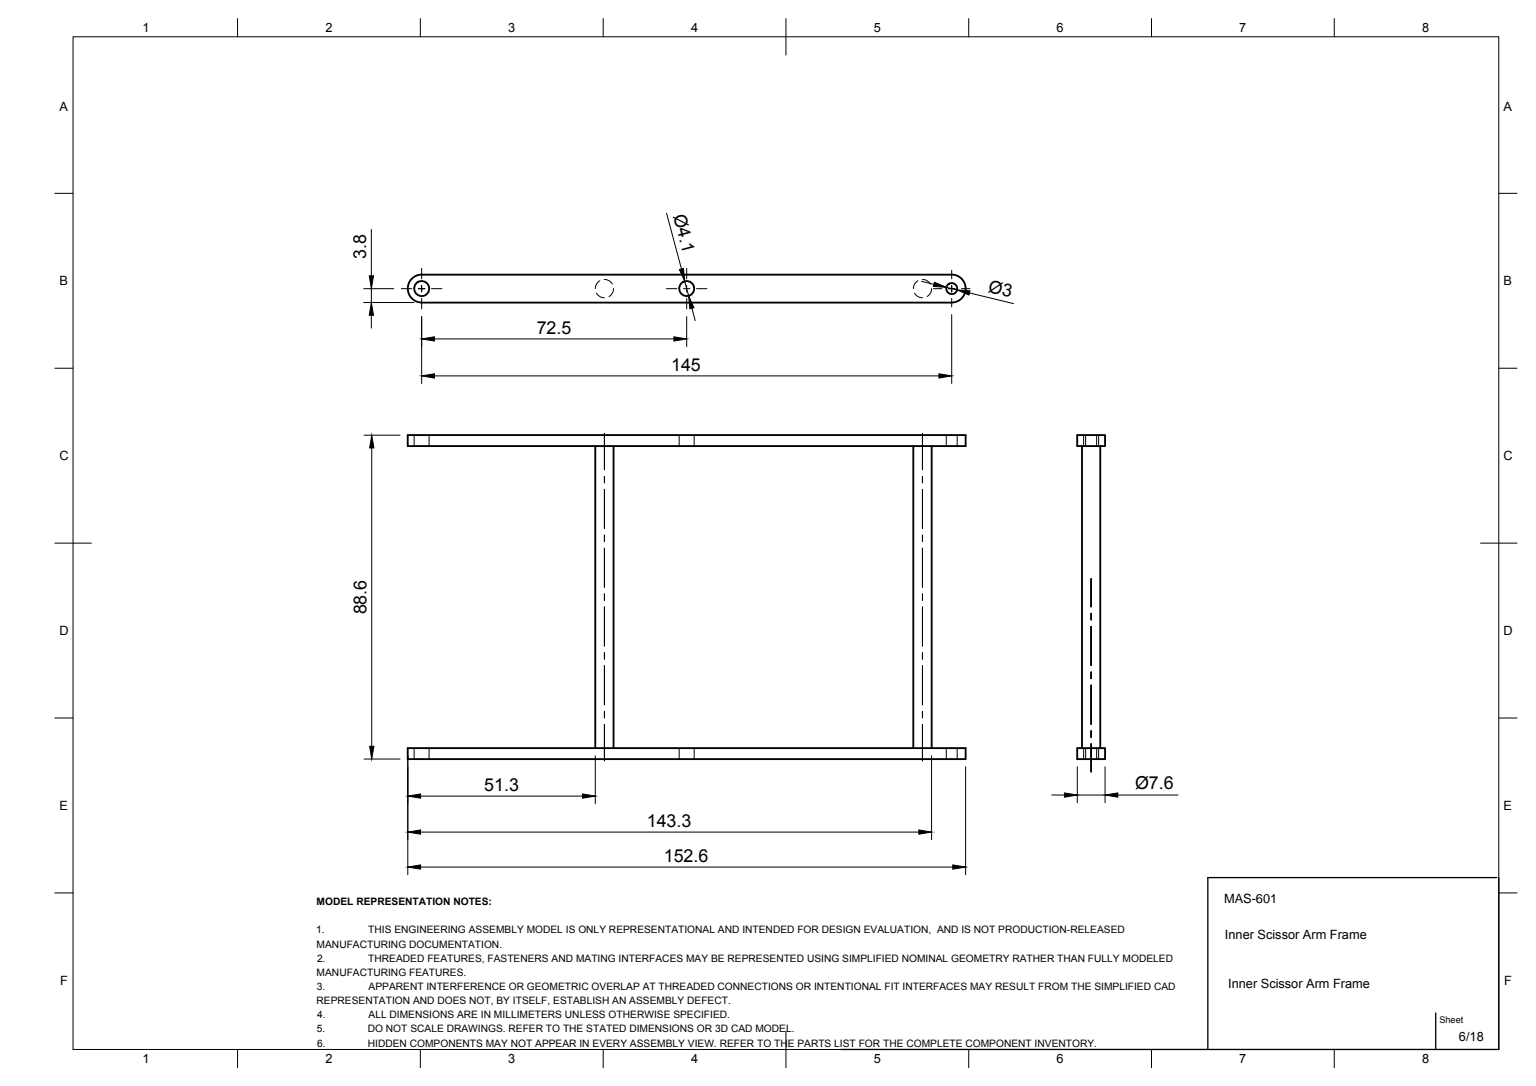
ISO-10303-21;
HEADER;
FILE_DESCRIPTION((''),'2;1');
FILE_NAME('Inner Scissor Arm Frame.step','2026-10-06T07:37:42+05:00',(''),(''),'','','');
FILE_SCHEMA (('AUTOMOTIVE_DESIGN { 1 0 10303 214 3 1 1 }'));
ENDSEC;
DATA;
#10=MECHANICAL_DESIGN_GEOMETRIC_PRESENTATION_REPRESENTATION('',(#376),#18757);
#342=SHAPE_REPRESENTATION_RELATIONSHIP('SRR','None',#18860,#359) ;
#359=ADVANCED_BREP_SHAPE_REPRESENTATION('',(#393),#18743) ;
#376=STYLED_ITEM('',(#18954),#393) ;
#393=MANIFOLD_SOLID_BREP('Inner Scissor Arm Frame',#9545) ;
#549=CYLINDRICAL_SURFACE('',#10026,2.5) ;
#550=CYLINDRICAL_SURFACE('',#10029,2.5) ;
#551=CYLINDRICAL_SURFACE('',#10032,2.05) ;
#552=CYLINDRICAL_SURFACE('',#10035,1.5) ;
#553=CYLINDRICAL_SURFACE('',#10038,2.05) ;
#554=CYLINDRICAL_SURFACE('',#10042,3.8) ;
#555=CYLINDRICAL_SURFACE('',#10046,3.8) ;
#556=CYLINDRICAL_SURFACE('',#10051,1.5) ;
#557=CYLINDRICAL_SURFACE('',#10054,2.05) ;
#558=CYLINDRICAL_SURFACE('',#10057,2.05) ;
#559=CYLINDRICAL_SURFACE('',#10061,3.8) ;
#560=CYLINDRICAL_SURFACE('',#10065,3.8) ;
#696=FACE_BOUND('',#1819,.T.) ;
#697=FACE_BOUND('',#1820,.T.) ;
#698=FACE_BOUND('',#1821,.T.) ;
#699=FACE_BOUND('',#1822,.T.) ;
#700=FACE_BOUND('',#1823,.T.) ;
#701=FACE_BOUND('',#1825,.T.) ;
#702=FACE_BOUND('',#1826,.T.) ;
#703=FACE_BOUND('',#1827,.T.) ;
#704=FACE_BOUND('',#1836,.T.) ;
#705=FACE_BOUND('',#1837,.T.) ;
#706=FACE_BOUND('',#1838,.T.) ;
#707=FACE_BOUND('',#1840,.T.) ;
#708=FACE_BOUND('',#1841,.T.) ;
#709=FACE_BOUND('',#1842,.T.) ;
#710=FACE_BOUND('',#1843,.T.) ;
#711=FACE_BOUND('',#1844,.T.) ;
#848=PLANE('',#10041) ;
#849=PLANE('',#10045) ;
#850=PLANE('',#10049) ;
#851=PLANE('',#10050) ;
#852=PLANE('',#10060) ;
#853=PLANE('',#10064) ;
#854=PLANE('',#10068) ;
#855=PLANE('',#10069) ;
#1245=FACE_OUTER_BOUND('',#1809,.T.) ;
#1246=FACE_OUTER_BOUND('',#1810,.T.) ;
#1247=FACE_OUTER_BOUND('',#1811,.T.) ;
#1248=FACE_OUTER_BOUND('',#1812,.T.) ;
#1249=FACE_OUTER_BOUND('',#1813,.T.) ;
#1250=FACE_OUTER_BOUND('',#1814,.T.) ;
#1251=FACE_OUTER_BOUND('',#1815,.T.) ;
#1252=FACE_OUTER_BOUND('',#1816,.T.) ;
#1253=FACE_OUTER_BOUND('',#1817,.T.) ;
#1254=FACE_OUTER_BOUND('',#1818,.T.) ;
#1255=FACE_OUTER_BOUND('',#1824,.T.) ;
#1256=FACE_OUTER_BOUND('',#1828,.T.) ;
#1257=FACE_OUTER_BOUND('',#1829,.T.) ;
#1258=FACE_OUTER_BOUND('',#1830,.T.) ;
#1259=FACE_OUTER_BOUND('',#1831,.T.) ;
#1260=FACE_OUTER_BOUND('',#1832,.T.) ;
#1261=FACE_OUTER_BOUND('',#1833,.T.) ;
#1262=FACE_OUTER_BOUND('',#1834,.T.) ;
#1263=FACE_OUTER_BOUND('',#1835,.T.) ;
#1264=FACE_OUTER_BOUND('',#1839,.T.) ;
#1809=EDGE_LOOP('',(#7161,#7162,#7163,#7164)) ;
#1810=EDGE_LOOP('',(#7165,#7166,#7167,#7168)) ;
#1811=EDGE_LOOP('',(#7169,#7170,#7171,#7172)) ;
#1812=EDGE_LOOP('',(#7173,#7174,#7175,#7176)) ;
#1813=EDGE_LOOP('',(#7177,#7178,#7179,#7180)) ;
#1814=EDGE_LOOP('',(#7181,#7182,#7183,#7184)) ;
#1815=EDGE_LOOP('',(#7185,#7186,#7187,#7188)) ;
#1816=EDGE_LOOP('',(#7189,#7190,#7191,#7192)) ;
#1817=EDGE_LOOP('',(#7193,#7194,#7195,#7196)) ;
#1818=EDGE_LOOP('',(#7197,#7198,#7199,#7200)) ;
#1819=EDGE_LOOP('',(#7201)) ;
#1820=EDGE_LOOP('',(#7202)) ;
#1821=EDGE_LOOP('',(#7203)) ;
#1822=EDGE_LOOP('',(#7204)) ;
#1823=EDGE_LOOP('',(#7205)) ;
#1824=EDGE_LOOP('',(#7206,#7207,#7208,#7209)) ;
#1825=EDGE_LOOP('',(#7210)) ;
#1826=EDGE_LOOP('',(#7211)) ;
#1827=EDGE_LOOP('',(#7212)) ;
#1828=EDGE_LOOP('',(#7213,#7214,#7215,#7216)) ;
#1829=EDGE_LOOP('',(#7217,#7218,#7219,#7220)) ;
#1830=EDGE_LOOP('',(#7221,#7222,#7223,#7224)) ;
#1831=EDGE_LOOP('',(#7225,#7226,#7227,#7228)) ;
#1832=EDGE_LOOP('',(#7229,#7230,#7231,#7232)) ;
#1833=EDGE_LOOP('',(#7233,#7234,#7235,#7236)) ;
#1834=EDGE_LOOP('',(#7237,#7238,#7239,#7240)) ;
#1835=EDGE_LOOP('',(#7241,#7242,#7243,#7244)) ;
#1836=EDGE_LOOP('',(#7245)) ;
#1837=EDGE_LOOP('',(#7246)) ;
#1838=EDGE_LOOP('',(#7247)) ;
#1839=EDGE_LOOP('',(#7248,#7249,#7250,#7251)) ;
#1840=EDGE_LOOP('',(#7252)) ;
#1841=EDGE_LOOP('',(#7253)) ;
#1842=EDGE_LOOP('',(#7254)) ;
#1843=EDGE_LOOP('',(#7255)) ;
#1844=EDGE_LOOP('',(#7256)) ;
#2514=LINE('',#14482,#3285) ;
#2515=LINE('',#14488,#3286) ;
#2516=LINE('',#14494,#3287) ;
#2517=LINE('',#14500,#3288) ;
#2518=LINE('',#14506,#3289) ;
#2519=LINE('',#14511,#3290) ;
#2520=LINE('',#14513,#3291) ;
#2521=LINE('',#14515,#3292) ;
#2522=LINE('',#14516,#3293) ;
#2523=LINE('',#14522,#3294) ;
#2524=LINE('',#14525,#3295) ;
#2525=LINE('',#14527,#3296) ;
#2526=LINE('',#14528,#3297) ;
#2527=LINE('',#14538,#3298) ;
#2528=LINE('',#14544,#3299) ;
#2529=LINE('',#14550,#3300) ;
#2530=LINE('',#14555,#3301) ;
#2531=LINE('',#14557,#3302) ;
#2532=LINE('',#14559,#3303) ;
#2533=LINE('',#14560,#3304) ;
#2534=LINE('',#14566,#3305) ;
#2535=LINE('',#14569,#3306) ;
#2536=LINE('',#14571,#3307) ;
#2537=LINE('',#14572,#3308) ;
#3285=VECTOR('',#11558,2.5) ;
#3286=VECTOR('',#11565,2.5) ;
#3287=VECTOR('',#11572,2.05) ;
#3288=VECTOR('',#11579,1.5) ;
#3289=VECTOR('',#11586,2.05) ;
#3290=VECTOR('',#11591,10.) ;
#3291=VECTOR('',#11592,10.) ;
#3292=VECTOR('',#11593,10.) ;
#3293=VECTOR('',#11594,10.) ;
#3294=VECTOR('',#11601,10.) ;
#3295=VECTOR('',#11604,10.) ;
#3296=VECTOR('',#11605,10.) ;
#3297=VECTOR('',#11606,10.) ;
#3298=VECTOR('',#11621,1.5) ;
#3299=VECTOR('',#11628,2.05) ;
#3300=VECTOR('',#11635,2.05) ;
#3301=VECTOR('',#11640,10.) ;
#3302=VECTOR('',#11641,10.) ;
#3303=VECTOR('',#11642,10.) ;
#3304=VECTOR('',#11643,10.) ;
#3305=VECTOR('',#11650,10.) ;
#3306=VECTOR('',#11653,10.) ;
#3307=VECTOR('',#11654,10.) ;
#3308=VECTOR('',#11655,10.) ;
#3891=CIRCLE('',#10027,2.5) ;
#3892=CIRCLE('',#10028,2.5) ;
#3893=CIRCLE('',#10030,2.5) ;
#3894=CIRCLE('',#10031,2.5) ;
#3895=CIRCLE('',#10033,2.05) ;
#3896=CIRCLE('',#10034,2.05) ;
#3897=CIRCLE('',#10036,1.5) ;
#3898=CIRCLE('',#10037,1.5) ;
#3899=CIRCLE('',#10039,2.05) ;
#3900=CIRCLE('',#10040,2.05) ;
#3901=CIRCLE('',#10043,3.8) ;
#3902=CIRCLE('',#10044,3.8) ;
#3903=CIRCLE('',#10047,3.8) ;
#3904=CIRCLE('',#10048,3.8) ;
#3905=CIRCLE('',#10052,1.5) ;
#3906=CIRCLE('',#10053,1.5) ;
#3907=CIRCLE('',#10055,2.05) ;
#3908=CIRCLE('',#10056,2.05) ;
#3909=CIRCLE('',#10058,2.05) ;
#3910=CIRCLE('',#10059,2.05) ;
#3911=CIRCLE('',#10062,3.8) ;
#3912=CIRCLE('',#10063,3.8) ;
#3913=CIRCLE('',#10066,3.8) ;
#3914=CIRCLE('',#10067,3.8) ;
#4418=VERTEX_POINT('',#14479) ;
#4419=VERTEX_POINT('',#14481) ;
#4420=VERTEX_POINT('',#14485) ;
#4421=VERTEX_POINT('',#14487) ;
#4422=VERTEX_POINT('',#14491) ;
#4423=VERTEX_POINT('',#14493) ;
#4424=VERTEX_POINT('',#14497) ;
#4425=VERTEX_POINT('',#14499) ;
#4426=VERTEX_POINT('',#14503) ;
#4427=VERTEX_POINT('',#14505) ;
#4428=VERTEX_POINT('',#14509) ;
#4429=VERTEX_POINT('',#14510) ;
#4430=VERTEX_POINT('',#14512) ;
#4431=VERTEX_POINT('',#14514) ;
#4432=VERTEX_POINT('',#14518) ;
#4433=VERTEX_POINT('',#14520) ;
#4434=VERTEX_POINT('',#14524) ;
#4435=VERTEX_POINT('',#14526) ;
#4436=VERTEX_POINT('',#14535) ;
#4437=VERTEX_POINT('',#14537) ;
#4438=VERTEX_POINT('',#14541) ;
#4439=VERTEX_POINT('',#14543) ;
#4440=VERTEX_POINT('',#14547) ;
#4441=VERTEX_POINT('',#14549) ;
#4442=VERTEX_POINT('',#14553) ;
#4443=VERTEX_POINT('',#14554) ;
#4444=VERTEX_POINT('',#14556) ;
#4445=VERTEX_POINT('',#14558) ;
#4446=VERTEX_POINT('',#14562) ;
#4447=VERTEX_POINT('',#14564) ;
#4448=VERTEX_POINT('',#14568) ;
#4449=VERTEX_POINT('',#14570) ;
#5427=EDGE_CURVE('',#4418,#4418,#3891,.T.) ;
#5428=EDGE_CURVE('',#4418,#4419,#2514,.T.) ;
#5429=EDGE_CURVE('',#4419,#4419,#3892,.T.) ;
#5430=EDGE_CURVE('',#4420,#4420,#3893,.T.) ;
#5431=EDGE_CURVE('',#4420,#4421,#2515,.T.) ;
#5432=EDGE_CURVE('',#4421,#4421,#3894,.T.) ;
#5433=EDGE_CURVE('',#4422,#4422,#3895,.T.) ;
#5434=EDGE_CURVE('',#4422,#4423,#2516,.T.) ;
#5435=EDGE_CURVE('',#4423,#4423,#3896,.T.) ;
#5436=EDGE_CURVE('',#4424,#4424,#3897,.T.) ;
#5437=EDGE_CURVE('',#4424,#4425,#2517,.T.) ;
#5438=EDGE_CURVE('',#4425,#4425,#3898,.T.) ;
#5439=EDGE_CURVE('',#4426,#4426,#3899,.T.) ;
#5440=EDGE_CURVE('',#4426,#4427,#2518,.T.) ;
#5441=EDGE_CURVE('',#4427,#4427,#3900,.T.) ;
#5442=EDGE_CURVE('',#4428,#4429,#2519,.T.) ;
#5443=EDGE_CURVE('',#4429,#4430,#2520,.T.) ;
#5444=EDGE_CURVE('',#4431,#4430,#2521,.T.) ;
#5445=EDGE_CURVE('',#4428,#4431,#2522,.T.) ;
#5446=EDGE_CURVE('',#4432,#4428,#3901,.T.) ;
#5447=EDGE_CURVE('',#4433,#4431,#3902,.T.) ;
#5448=EDGE_CURVE('',#4432,#4433,#2523,.T.) ;
#5449=EDGE_CURVE('',#4434,#4432,#2524,.T.) ;
#5450=EDGE_CURVE('',#4435,#4433,#2525,.T.) ;
#5451=EDGE_CURVE('',#4434,#4435,#2526,.T.) ;
#5452=EDGE_CURVE('',#4429,#4434,#3903,.T.) ;
#5453=EDGE_CURVE('',#4430,#4435,#3904,.T.) ;
#5454=EDGE_CURVE('',#4436,#4436,#3905,.T.) ;
#5455=EDGE_CURVE('',#4436,#4437,#2527,.T.) ;
#5456=EDGE_CURVE('',#4437,#4437,#3906,.T.) ;
#5457=EDGE_CURVE('',#4438,#4438,#3907,.T.) ;
#5458=EDGE_CURVE('',#4438,#4439,#2528,.T.) ;
#5459=EDGE_CURVE('',#4439,#4439,#3908,.T.) ;
#5460=EDGE_CURVE('',#4440,#4440,#3909,.T.) ;
#5461=EDGE_CURVE('',#4440,#4441,#2529,.T.) ;
#5462=EDGE_CURVE('',#4441,#4441,#3910,.T.) ;
#5463=EDGE_CURVE('',#4442,#4443,#2530,.T.) ;
#5464=EDGE_CURVE('',#4443,#4444,#2531,.T.) ;
#5465=EDGE_CURVE('',#4445,#4444,#2532,.T.) ;
#5466=EDGE_CURVE('',#4442,#4445,#2533,.T.) ;
#5467=EDGE_CURVE('',#4446,#4442,#3911,.T.) ;
#5468=EDGE_CURVE('',#4447,#4445,#3912,.T.) ;
#5469=EDGE_CURVE('',#4446,#4447,#2534,.T.) ;
#5470=EDGE_CURVE('',#4448,#4446,#2535,.T.) ;
#5471=EDGE_CURVE('',#4449,#4447,#2536,.T.) ;
#5472=EDGE_CURVE('',#4448,#4449,#2537,.T.) ;
#5473=EDGE_CURVE('',#4443,#4448,#3913,.T.) ;
#5474=EDGE_CURVE('',#4444,#4449,#3914,.T.) ;
#7161=ORIENTED_EDGE('',*,*,#5427,.F.) ;
#7162=ORIENTED_EDGE('',*,*,#5428,.T.) ;
#7163=ORIENTED_EDGE('',*,*,#5429,.F.) ;
#7164=ORIENTED_EDGE('',*,*,#5428,.F.) ;
#7165=ORIENTED_EDGE('',*,*,#5430,.F.) ;
#7166=ORIENTED_EDGE('',*,*,#5431,.T.) ;
#7167=ORIENTED_EDGE('',*,*,#5432,.F.) ;
#7168=ORIENTED_EDGE('',*,*,#5431,.F.) ;
#7169=ORIENTED_EDGE('',*,*,#5433,.F.) ;
#7170=ORIENTED_EDGE('',*,*,#5434,.T.) ;
#7171=ORIENTED_EDGE('',*,*,#5435,.T.) ;
#7172=ORIENTED_EDGE('',*,*,#5434,.F.) ;
#7173=ORIENTED_EDGE('',*,*,#5436,.F.) ;
#7174=ORIENTED_EDGE('',*,*,#5437,.T.) ;
#7175=ORIENTED_EDGE('',*,*,#5438,.T.) ;
#7176=ORIENTED_EDGE('',*,*,#5437,.F.) ;
#7177=ORIENTED_EDGE('',*,*,#5439,.F.) ;
#7178=ORIENTED_EDGE('',*,*,#5440,.T.) ;
#7179=ORIENTED_EDGE('',*,*,#5441,.T.) ;
#7180=ORIENTED_EDGE('',*,*,#5440,.F.) ;
#7181=ORIENTED_EDGE('',*,*,#5442,.T.) ;
#7182=ORIENTED_EDGE('',*,*,#5443,.T.) ;
#7183=ORIENTED_EDGE('',*,*,#5444,.F.) ;
#7184=ORIENTED_EDGE('',*,*,#5445,.F.) ;
#7185=ORIENTED_EDGE('',*,*,#5446,.T.) ;
#7186=ORIENTED_EDGE('',*,*,#5445,.T.) ;
#7187=ORIENTED_EDGE('',*,*,#5447,.F.) ;
#7188=ORIENTED_EDGE('',*,*,#5448,.F.) ;
#7189=ORIENTED_EDGE('',*,*,#5449,.T.) ;
#7190=ORIENTED_EDGE('',*,*,#5448,.T.) ;
#7191=ORIENTED_EDGE('',*,*,#5450,.F.) ;
#7192=ORIENTED_EDGE('',*,*,#5451,.F.) ;
#7193=ORIENTED_EDGE('',*,*,#5452,.T.) ;
#7194=ORIENTED_EDGE('',*,*,#5451,.T.) ;
#7195=ORIENTED_EDGE('',*,*,#5453,.F.) ;
#7196=ORIENTED_EDGE('',*,*,#5443,.F.) ;
#7197=ORIENTED_EDGE('',*,*,#5453,.T.) ;
#7198=ORIENTED_EDGE('',*,*,#5450,.T.) ;
#7199=ORIENTED_EDGE('',*,*,#5447,.T.) ;
#7200=ORIENTED_EDGE('',*,*,#5444,.T.) ;
#7201=ORIENTED_EDGE('',*,*,#5429,.T.) ;
#7202=ORIENTED_EDGE('',*,*,#5432,.T.) ;
#7203=ORIENTED_EDGE('',*,*,#5439,.T.) ;
#7204=ORIENTED_EDGE('',*,*,#5436,.T.) ;
#7205=ORIENTED_EDGE('',*,*,#5433,.T.) ;
#7206=ORIENTED_EDGE('',*,*,#5452,.F.) ;
#7207=ORIENTED_EDGE('',*,*,#5442,.F.) ;
#7208=ORIENTED_EDGE('',*,*,#5446,.F.) ;
#7209=ORIENTED_EDGE('',*,*,#5449,.F.) ;
#7210=ORIENTED_EDGE('',*,*,#5441,.F.) ;
#7211=ORIENTED_EDGE('',*,*,#5438,.F.) ;
#7212=ORIENTED_EDGE('',*,*,#5435,.F.) ;
#7213=ORIENTED_EDGE('',*,*,#5454,.F.) ;
#7214=ORIENTED_EDGE('',*,*,#5455,.T.) ;
#7215=ORIENTED_EDGE('',*,*,#5456,.T.) ;
#7216=ORIENTED_EDGE('',*,*,#5455,.F.) ;
#7217=ORIENTED_EDGE('',*,*,#5457,.F.) ;
#7218=ORIENTED_EDGE('',*,*,#5458,.T.) ;
#7219=ORIENTED_EDGE('',*,*,#5459,.T.) ;
#7220=ORIENTED_EDGE('',*,*,#5458,.F.) ;
#7221=ORIENTED_EDGE('',*,*,#5460,.F.) ;
#7222=ORIENTED_EDGE('',*,*,#5461,.T.) ;
#7223=ORIENTED_EDGE('',*,*,#5462,.T.) ;
#7224=ORIENTED_EDGE('',*,*,#5461,.F.) ;
#7225=ORIENTED_EDGE('',*,*,#5463,.T.) ;
#7226=ORIENTED_EDGE('',*,*,#5464,.T.) ;
#7227=ORIENTED_EDGE('',*,*,#5465,.F.) ;
#7228=ORIENTED_EDGE('',*,*,#5466,.F.) ;
#7229=ORIENTED_EDGE('',*,*,#5467,.T.) ;
#7230=ORIENTED_EDGE('',*,*,#5466,.T.) ;
#7231=ORIENTED_EDGE('',*,*,#5468,.F.) ;
#7232=ORIENTED_EDGE('',*,*,#5469,.F.) ;
#7233=ORIENTED_EDGE('',*,*,#5470,.T.) ;
#7234=ORIENTED_EDGE('',*,*,#5469,.T.) ;
#7235=ORIENTED_EDGE('',*,*,#5471,.F.) ;
#7236=ORIENTED_EDGE('',*,*,#5472,.F.) ;
#7237=ORIENTED_EDGE('',*,*,#5473,.T.) ;
#7238=ORIENTED_EDGE('',*,*,#5472,.T.) ;
#7239=ORIENTED_EDGE('',*,*,#5474,.F.) ;
#7240=ORIENTED_EDGE('',*,*,#5464,.F.) ;
#7241=ORIENTED_EDGE('',*,*,#5474,.T.) ;
#7242=ORIENTED_EDGE('',*,*,#5471,.T.) ;
#7243=ORIENTED_EDGE('',*,*,#5468,.T.) ;
#7244=ORIENTED_EDGE('',*,*,#5465,.T.) ;
#7245=ORIENTED_EDGE('',*,*,#5460,.T.) ;
#7246=ORIENTED_EDGE('',*,*,#5457,.T.) ;
#7247=ORIENTED_EDGE('',*,*,#5454,.T.) ;
#7248=ORIENTED_EDGE('',*,*,#5473,.F.) ;
#7249=ORIENTED_EDGE('',*,*,#5463,.F.) ;
#7250=ORIENTED_EDGE('',*,*,#5467,.F.) ;
#7251=ORIENTED_EDGE('',*,*,#5470,.F.) ;
#7252=ORIENTED_EDGE('',*,*,#5427,.T.) ;
#7253=ORIENTED_EDGE('',*,*,#5430,.T.) ;
#7254=ORIENTED_EDGE('',*,*,#5462,.F.) ;
#7255=ORIENTED_EDGE('',*,*,#5459,.F.) ;
#7256=ORIENTED_EDGE('',*,*,#5456,.F.) ;
#9181=ADVANCED_FACE('',(#1245),#549,.T.) ;
#9182=ADVANCED_FACE('',(#1246),#550,.T.) ;
#9183=ADVANCED_FACE('',(#1247),#551,.F.) ;
#9184=ADVANCED_FACE('',(#1248),#552,.F.) ;
#9185=ADVANCED_FACE('',(#1249),#553,.F.) ;
#9186=ADVANCED_FACE('',(#1250),#848,.T.) ;
#9187=ADVANCED_FACE('',(#1251),#554,.T.) ;
#9188=ADVANCED_FACE('',(#1252),#849,.T.) ;
#9189=ADVANCED_FACE('',(#1253),#555,.T.) ;
#9190=ADVANCED_FACE('',(#1254,#696,#697,#698,#699,#700),#850,.T.) ;
#9191=ADVANCED_FACE('',(#1255,#701,#702,#703),#851,.F.) ;
#9192=ADVANCED_FACE('',(#1256),#556,.F.) ;
#9193=ADVANCED_FACE('',(#1257),#557,.F.) ;
#9194=ADVANCED_FACE('',(#1258),#558,.F.) ;
#9195=ADVANCED_FACE('',(#1259),#852,.T.) ;
#9196=ADVANCED_FACE('',(#1260),#559,.T.) ;
#9197=ADVANCED_FACE('',(#1261),#853,.T.) ;
#9198=ADVANCED_FACE('',(#1262),#560,.T.) ;
#9199=ADVANCED_FACE('',(#1263,#704,#705,#706),#854,.T.) ;
#9200=ADVANCED_FACE('',(#1264,#707,#708,#709,#710,#711),#855,.F.) ;
#9545=CLOSED_SHELL('',(#9181,#9182,#9183,#9184,#9185,#9186,#9187,#9188,
#9189,#9190,#9191,#9192,#9193,#9194,#9195,#9196,#9197,#9198,#9199,#9200)) ;
#10025=AXIS2_PLACEMENT_3D('',#14477,#11552,#11553) ;
#10026=AXIS2_PLACEMENT_3D('',#14478,#11554,#11555) ;
#10027=AXIS2_PLACEMENT_3D('',#14480,#11556,#11557) ;
#10028=AXIS2_PLACEMENT_3D('',#14483,#11559,#11560) ;
#10029=AXIS2_PLACEMENT_3D('',#14484,#11561,#11562) ;
#10030=AXIS2_PLACEMENT_3D('',#14486,#11563,#11564) ;
#10031=AXIS2_PLACEMENT_3D('',#14489,#11566,#11567) ;
#10032=AXIS2_PLACEMENT_3D('',#14490,#11568,#11569) ;
#10033=AXIS2_PLACEMENT_3D('',#14492,#11570,#11571) ;
#10034=AXIS2_PLACEMENT_3D('',#14495,#11573,#11574) ;
#10035=AXIS2_PLACEMENT_3D('',#14496,#11575,#11576) ;
#10036=AXIS2_PLACEMENT_3D('',#14498,#11577,#11578) ;
#10037=AXIS2_PLACEMENT_3D('',#14501,#11580,#11581) ;
#10038=AXIS2_PLACEMENT_3D('',#14502,#11582,#11583) ;
#10039=AXIS2_PLACEMENT_3D('',#14504,#11584,#11585) ;
#10040=AXIS2_PLACEMENT_3D('',#14507,#11587,#11588) ;
#10041=AXIS2_PLACEMENT_3D('',#14508,#11589,#11590) ;
#10042=AXIS2_PLACEMENT_3D('',#14517,#11595,#11596) ;
#10043=AXIS2_PLACEMENT_3D('',#14519,#11597,#11598) ;
#10044=AXIS2_PLACEMENT_3D('',#14521,#11599,#11600) ;
#10045=AXIS2_PLACEMENT_3D('',#14523,#11602,#11603) ;
#10046=AXIS2_PLACEMENT_3D('',#14529,#11607,#11608) ;
#10047=AXIS2_PLACEMENT_3D('',#14530,#11609,#11610) ;
#10048=AXIS2_PLACEMENT_3D('',#14531,#11611,#11612) ;
#10049=AXIS2_PLACEMENT_3D('',#14532,#11613,#11614) ;
#10050=AXIS2_PLACEMENT_3D('',#14533,#11615,#11616) ;
#10051=AXIS2_PLACEMENT_3D('',#14534,#11617,#11618) ;
#10052=AXIS2_PLACEMENT_3D('',#14536,#11619,#11620) ;
#10053=AXIS2_PLACEMENT_3D('',#14539,#11622,#11623) ;
#10054=AXIS2_PLACEMENT_3D('',#14540,#11624,#11625) ;
#10055=AXIS2_PLACEMENT_3D('',#14542,#11626,#11627) ;
#10056=AXIS2_PLACEMENT_3D('',#14545,#11629,#11630) ;
#10057=AXIS2_PLACEMENT_3D('',#14546,#11631,#11632) ;
#10058=AXIS2_PLACEMENT_3D('',#14548,#11633,#11634) ;
#10059=AXIS2_PLACEMENT_3D('',#14551,#11636,#11637) ;
#10060=AXIS2_PLACEMENT_3D('',#14552,#11638,#11639) ;
#10061=AXIS2_PLACEMENT_3D('',#14561,#11644,#11645) ;
#10062=AXIS2_PLACEMENT_3D('',#14563,#11646,#11647) ;
#10063=AXIS2_PLACEMENT_3D('',#14565,#11648,#11649) ;
#10064=AXIS2_PLACEMENT_3D('',#14567,#11651,#11652) ;
#10065=AXIS2_PLACEMENT_3D('',#14573,#11656,#11657) ;
#10066=AXIS2_PLACEMENT_3D('',#14574,#11658,#11659) ;
#10067=AXIS2_PLACEMENT_3D('',#14575,#11660,#11661) ;
#10068=AXIS2_PLACEMENT_3D('',#14576,#11662,#11663) ;
#10069=AXIS2_PLACEMENT_3D('',#14577,#11664,#11665) ;
#11552=DIRECTION('axis',(0.,0.,1.)) ;
#11553=DIRECTION('refdir',(1.,0.,0.)) ;
#11554=DIRECTION('center_axis',(0.,1.,0.)) ;
#11555=DIRECTION('ref_axis',(1.,0.,0.)) ;
#11556=DIRECTION('center_axis',(0.,1.,0.)) ;
#11557=DIRECTION('ref_axis',(1.,0.,0.)) ;
#11558=DIRECTION('',(0.,-1.,0.)) ;
#11559=DIRECTION('center_axis',(0.,-1.,0.)) ;
#11560=DIRECTION('ref_axis',(1.,0.,0.)) ;
#11561=DIRECTION('center_axis',(0.,1.,0.)) ;
#11562=DIRECTION('ref_axis',(1.,0.,0.)) ;
#11563=DIRECTION('center_axis',(0.,1.,0.)) ;
#11564=DIRECTION('ref_axis',(1.,0.,0.)) ;
#11565=DIRECTION('',(0.,-1.,0.)) ;
#11566=DIRECTION('center_axis',(0.,-1.,0.)) ;
#11567=DIRECTION('ref_axis',(1.,0.,0.)) ;
#11568=DIRECTION('center_axis',(0.,1.,0.)) ;
#11569=DIRECTION('ref_axis',(1.,0.,0.)) ;
#11570=DIRECTION('center_axis',(0.,-1.,0.)) ;
#11571=DIRECTION('ref_axis',(1.,0.,0.)) ;
#11572=DIRECTION('',(0.,-1.,0.)) ;
#11573=DIRECTION('center_axis',(0.,-1.,0.)) ;
#11574=DIRECTION('ref_axis',(1.,0.,0.)) ;
#11575=DIRECTION('center_axis',(0.,1.,0.)) ;
#11576=DIRECTION('ref_axis',(1.,0.,0.)) ;
#11577=DIRECTION('center_axis',(0.,-1.,0.)) ;
#11578=DIRECTION('ref_axis',(1.,0.,0.)) ;
#11579=DIRECTION('',(0.,-1.,0.)) ;
#11580=DIRECTION('center_axis',(0.,-1.,0.)) ;
#11581=DIRECTION('ref_axis',(1.,0.,0.)) ;
#11582=DIRECTION('center_axis',(0.,1.,0.)) ;
#11583=DIRECTION('ref_axis',(1.,0.,0.)) ;
#11584=DIRECTION('center_axis',(0.,-1.,0.)) ;
#11585=DIRECTION('ref_axis',(1.,0.,0.)) ;
#11586=DIRECTION('',(0.,-1.,0.)) ;
#11587=DIRECTION('center_axis',(0.,-1.,0.)) ;
#11588=DIRECTION('ref_axis',(1.,0.,0.)) ;
#11589=DIRECTION('center_axis',(-0.0648275862068965,0.,0.997896479634329)) ;
#11590=DIRECTION('ref_axis',(0.997896479634329,0.,0.0648275862068965)) ;
#11591=DIRECTION('',(0.997896479634329,0.,0.0648275862068965)) ;
#11592=DIRECTION('',(0.,1.,0.)) ;
#11593=DIRECTION('',(0.997896479634329,0.,0.0648275862068965)) ;
#11594=DIRECTION('',(0.,1.,0.)) ;
#11595=DIRECTION('center_axis',(0.,1.,0.)) ;
#11596=DIRECTION('ref_axis',(0.0648275862068983,0.,-0.997896479634329)) ;
#11597=DIRECTION('center_axis',(0.,1.,0.)) ;
#11598=DIRECTION('ref_axis',(0.0648275862068983,0.,-0.997896479634329)) ;
#11599=DIRECTION('center_axis',(0.,1.,0.)) ;
#11600=DIRECTION('ref_axis',(0.0648275862068983,0.,-0.997896479634329)) ;
#11601=DIRECTION('',(0.,1.,0.)) ;
#11602=DIRECTION('center_axis',(0.0648275862068965,0.,-0.997896479634329)) ;
#11603=DIRECTION('ref_axis',(-0.997896479634329,0.,-0.0648275862068965)) ;
#11604=DIRECTION('',(-0.997896479634329,0.,-0.0648275862068965)) ;
#11605=DIRECTION('',(-0.997896479634329,0.,-0.0648275862068965)) ;
#11606=DIRECTION('',(0.,1.,0.)) ;
#11607=DIRECTION('center_axis',(0.,1.,0.)) ;
#11608=DIRECTION('ref_axis',(-0.0648275862069006,0.,0.997896479634329)) ;
#11609=DIRECTION('center_axis',(0.,1.,0.)) ;
#11610=DIRECTION('ref_axis',(-0.0648275862069006,0.,0.997896479634329)) ;
#11611=DIRECTION('center_axis',(0.,1.,0.)) ;
#11612=DIRECTION('ref_axis',(-0.0648275862069006,0.,0.997896479634329)) ;
#11613=DIRECTION('center_axis',(0.,1.,0.)) ;
#11614=DIRECTION('ref_axis',(1.,0.,0.)) ;
#11615=DIRECTION('center_axis',(0.,1.,0.)) ;
#11616=DIRECTION('ref_axis',(1.,0.,0.)) ;
#11617=DIRECTION('center_axis',(0.,1.,0.)) ;
#11618=DIRECTION('ref_axis',(1.,0.,0.)) ;
#11619=DIRECTION('center_axis',(0.,-1.,0.)) ;
#11620=DIRECTION('ref_axis',(1.,0.,0.)) ;
#11621=DIRECTION('',(0.,-1.,0.)) ;
#11622=DIRECTION('center_axis',(0.,-1.,0.)) ;
#11623=DIRECTION('ref_axis',(1.,0.,0.)) ;
#11624=DIRECTION('center_axis',(0.,1.,0.)) ;
#11625=DIRECTION('ref_axis',(1.,0.,0.)) ;
#11626=DIRECTION('center_axis',(0.,-1.,0.)) ;
#11627=DIRECTION('ref_axis',(1.,0.,0.)) ;
#11628=DIRECTION('',(0.,-1.,0.)) ;
#11629=DIRECTION('center_axis',(0.,-1.,0.)) ;
#11630=DIRECTION('ref_axis',(1.,0.,0.)) ;
#11631=DIRECTION('center_axis',(0.,1.,0.)) ;
#11632=DIRECTION('ref_axis',(1.,0.,0.)) ;
#11633=DIRECTION('center_axis',(0.,-1.,0.)) ;
#11634=DIRECTION('ref_axis',(1.,0.,0.)) ;
#11635=DIRECTION('',(0.,-1.,0.)) ;
#11636=DIRECTION('center_axis',(0.,-1.,0.)) ;
#11637=DIRECTION('ref_axis',(1.,0.,0.)) ;
#11638=DIRECTION('center_axis',(-0.0648275862068965,0.,0.997896479634329)) ;
#11639=DIRECTION('ref_axis',(0.997896479634329,0.,0.0648275862068965)) ;
#11640=DIRECTION('',(0.997896479634329,0.,0.0648275862068965)) ;
#11641=DIRECTION('',(0.,1.,0.)) ;
#11642=DIRECTION('',(0.997896479634329,0.,0.0648275862068965)) ;
#11643=DIRECTION('',(0.,1.,0.)) ;
#11644=DIRECTION('center_axis',(0.,1.,0.)) ;
#11645=DIRECTION('ref_axis',(0.0648275862068983,0.,-0.997896479634329)) ;
#11646=DIRECTION('center_axis',(0.,1.,0.)) ;
#11647=DIRECTION('ref_axis',(0.0648275862068983,0.,-0.997896479634329)) ;
#11648=DIRECTION('center_axis',(0.,1.,0.)) ;
#11649=DIRECTION('ref_axis',(0.0648275862068983,0.,-0.997896479634329)) ;
#11650=DIRECTION('',(0.,1.,0.)) ;
#11651=DIRECTION('center_axis',(0.0648275862068965,0.,-0.997896479634329)) ;
#11652=DIRECTION('ref_axis',(-0.997896479634329,0.,-0.0648275862068965)) ;
#11653=DIRECTION('',(-0.997896479634329,0.,-0.0648275862068965)) ;
#11654=DIRECTION('',(-0.997896479634329,0.,-0.0648275862068965)) ;
#11655=DIRECTION('',(0.,1.,0.)) ;
#11656=DIRECTION('center_axis',(0.,1.,0.)) ;
#11657=DIRECTION('ref_axis',(-0.0648275862069006,0.,0.997896479634329)) ;
#11658=DIRECTION('center_axis',(0.,1.,0.)) ;
#11659=DIRECTION('ref_axis',(-0.0648275862069006,0.,0.997896479634329)) ;
#11660=DIRECTION('center_axis',(0.,1.,0.)) ;
#11661=DIRECTION('ref_axis',(-0.0648275862069006,0.,0.997896479634329)) ;
#11662=DIRECTION('center_axis',(0.,1.,0.)) ;
#11663=DIRECTION('ref_axis',(1.,0.,0.)) ;
#11664=DIRECTION('center_axis',(0.,1.,0.)) ;
#11665=DIRECTION('ref_axis',(1.,0.,0.)) ;
#14477=CARTESIAN_POINT('',(0.,0.,0.)) ;
#14478=CARTESIAN_POINT('Origin',(22.1051760182835,-41.8,41.1586206896552)) ;
#14479=CARTESIAN_POINT('',(19.6051760182835,41.3,41.1586206896552)) ;
#14480=CARTESIAN_POINT('Origin',(22.1051760182835,41.3,41.1586206896552)) ;
#14481=CARTESIAN_POINT('',(19.6051760182835,-41.3,41.1586206896552)) ;
#14482=CARTESIAN_POINT('',(19.6051760182835,-41.8,41.1586206896552)) ;
#14483=CARTESIAN_POINT('Origin',(22.1051760182835,-41.3,41.1586206896552)) ;
#14484=CARTESIAN_POINT('Origin',(-64.7118177099031,-41.8,35.5186206896552)) ;
#14485=CARTESIAN_POINT('',(-67.2118177099031,41.3,35.5186206896552)) ;
#14486=CARTESIAN_POINT('Origin',(-64.7118177099031,41.3,35.5186206896552)) ;
#14487=CARTESIAN_POINT('',(-67.2118177099031,-41.3,35.5186206896552)) ;
#14488=CARTESIAN_POINT('',(-67.2118177099031,-41.8,35.5186206896552)) ;
#14489=CARTESIAN_POINT('Origin',(-64.7118177099031,-41.3,35.5186206896552)) ;
#14490=CARTESIAN_POINT('Origin',(72.,-44.3,44.4)) ;
#14491=CARTESIAN_POINT('',(69.95,-41.3,44.4)) ;
#14492=CARTESIAN_POINT('Origin',(72.,-41.3,44.4)) ;
#14493=CARTESIAN_POINT('',(69.95,-44.3,44.4)) ;
#14494=CARTESIAN_POINT('',(69.95,-44.3,44.4)) ;
#14495=CARTESIAN_POINT('Origin',(72.,-44.3,44.4)) ;
#14496=CARTESIAN_POINT('Origin',(-72.6949895469778,-44.3,35.)) ;
#14497=CARTESIAN_POINT('',(-74.1949895469778,-41.3,35.)) ;
#14498=CARTESIAN_POINT('Origin',(-72.6949895469778,-41.3,35.)) ;
#14499=CARTESIAN_POINT('',(-74.1949895469778,-44.3,35.)) ;
#14500=CARTESIAN_POINT('',(-74.1949895469778,-44.3,35.)) ;
#14501=CARTESIAN_POINT('Origin',(-72.6949895469778,-44.3,35.)) ;
#14502=CARTESIAN_POINT('Origin',(-0.347494773488876,-44.3,39.7)) ;
#14503=CARTESIAN_POINT('',(-2.39749477348888,-41.3,39.7)) ;
#14504=CARTESIAN_POINT('Origin',(-0.347494773488876,-41.3,39.7)) ;
#14505=CARTESIAN_POINT('',(-2.39749477348888,-44.3,39.7)) ;
#14506=CARTESIAN_POINT('',(-2.39749477348888,-44.3,39.7)) ;
#14507=CARTESIAN_POINT('Origin',(-0.347494773488876,-44.3,39.7)) ;
#14508=CARTESIAN_POINT('Origin',(-72.941334374564,-44.3,38.7920066226105)) ;
#14509=CARTESIAN_POINT('',(-72.941334374564,-44.3,38.7920066226105)) ;
#14510=CARTESIAN_POINT('',(71.7536551724138,-44.3,48.1920066226104)) ;
#14511=CARTESIAN_POINT('',(-72.941334374564,-44.3,38.7920066226105)) ;
#14512=CARTESIAN_POINT('',(71.7536551724138,-41.3,48.1920066226104)) ;
#14513=CARTESIAN_POINT('',(71.7536551724138,-44.3,48.1920066226104)) ;
#14514=CARTESIAN_POINT('',(-72.941334374564,-41.3,38.7920066226105)) ;
#14515=CARTESIAN_POINT('',(-72.941334374564,-41.3,38.7920066226105)) ;
#14516=CARTESIAN_POINT('',(-72.941334374564,-44.3,38.7920066226105)) ;
#14517=CARTESIAN_POINT('Origin',(-72.6949895469778,-44.3,35.)) ;
#14518=CARTESIAN_POINT('',(-72.4486447193915,-44.3,31.2079933773895)) ;
#14519=CARTESIAN_POINT('Origin',(-72.6949895469778,-44.3,35.)) ;
#14520=CARTESIAN_POINT('',(-72.4486447193915,-41.3,31.2079933773895)) ;
#14521=CARTESIAN_POINT('Origin',(-72.6949895469778,-41.3,35.)) ;
#14522=CARTESIAN_POINT('',(-72.4486447193915,-44.3,31.2079933773895)) ;
#14523=CARTESIAN_POINT('Origin',(72.2463448275862,-44.3,40.6079933773895)) ;
#14524=CARTESIAN_POINT('',(72.2463448275862,-44.3,40.6079933773895)) ;
#14525=CARTESIAN_POINT('',(72.2463448275862,-44.3,40.6079933773895)) ;
#14526=CARTESIAN_POINT('',(72.2463448275862,-41.3,40.6079933773895)) ;
#14527=CARTESIAN_POINT('',(72.2463448275862,-41.3,40.6079933773895)) ;
#14528=CARTESIAN_POINT('',(72.2463448275862,-44.3,40.6079933773895)) ;
#14529=CARTESIAN_POINT('Origin',(72.,-44.3,44.4)) ;
#14530=CARTESIAN_POINT('Origin',(72.,-44.3,44.4)) ;
#14531=CARTESIAN_POINT('Origin',(72.,-41.3,44.4)) ;
#14532=CARTESIAN_POINT('Origin',(-0.347494773488863,-41.3,39.7)) ;
#14533=CARTESIAN_POINT('Origin',(-0.347494773488863,-44.3,39.7)) ;
#14534=CARTESIAN_POINT('Origin',(-72.6949895469778,41.3,35.)) ;
#14535=CARTESIAN_POINT('',(-74.1949895469778,44.3,35.)) ;
#14536=CARTESIAN_POINT('Origin',(-72.6949895469778,44.3,35.)) ;
#14537=CARTESIAN_POINT('',(-74.1949895469778,41.3,35.)) ;
#14538=CARTESIAN_POINT('',(-74.1949895469778,41.3,35.)) ;
#14539=CARTESIAN_POINT('Origin',(-72.6949895469778,41.3,35.)) ;
#14540=CARTESIAN_POINT('Origin',(72.,41.3,44.4)) ;
#14541=CARTESIAN_POINT('',(69.95,44.3,44.4)) ;
#14542=CARTESIAN_POINT('Origin',(72.,44.3,44.4)) ;
#14543=CARTESIAN_POINT('',(69.95,41.3,44.4)) ;
#14544=CARTESIAN_POINT('',(69.95,41.3,44.4)) ;
#14545=CARTESIAN_POINT('Origin',(72.,41.3,44.4)) ;
#14546=CARTESIAN_POINT('Origin',(-0.347494773488876,41.3,39.7)) ;
#14547=CARTESIAN_POINT('',(-2.39749477348888,44.3,39.7)) ;
#14548=CARTESIAN_POINT('Origin',(-0.347494773488876,44.3,39.7)) ;
#14549=CARTESIAN_POINT('',(-2.39749477348888,41.3,39.7)) ;
#14550=CARTESIAN_POINT('',(-2.39749477348888,41.3,39.7)) ;
#14551=CARTESIAN_POINT('Origin',(-0.347494773488876,41.3,39.7)) ;
#14552=CARTESIAN_POINT('Origin',(-72.941334374564,41.3,38.7920066226105)) ;
#14553=CARTESIAN_POINT('',(-72.941334374564,41.3,38.7920066226105)) ;
#14554=CARTESIAN_POINT('',(71.7536551724138,41.3,48.1920066226104)) ;
#14555=CARTESIAN_POINT('',(-72.941334374564,41.3,38.7920066226105)) ;
#14556=CARTESIAN_POINT('',(71.7536551724138,44.3,48.1920066226104)) ;
#14557=CARTESIAN_POINT('',(71.7536551724138,41.3,48.1920066226104)) ;
#14558=CARTESIAN_POINT('',(-72.941334374564,44.3,38.7920066226105)) ;
#14559=CARTESIAN_POINT('',(-72.941334374564,44.3,38.7920066226105)) ;
#14560=CARTESIAN_POINT('',(-72.941334374564,41.3,38.7920066226105)) ;
#14561=CARTESIAN_POINT('Origin',(-72.6949895469778,41.3,35.)) ;
#14562=CARTESIAN_POINT('',(-72.4486447193915,41.3,31.2079933773895)) ;
#14563=CARTESIAN_POINT('Origin',(-72.6949895469778,41.3,35.)) ;
#14564=CARTESIAN_POINT('',(-72.4486447193915,44.3,31.2079933773895)) ;
#14565=CARTESIAN_POINT('Origin',(-72.6949895469778,44.3,35.)) ;
#14566=CARTESIAN_POINT('',(-72.4486447193915,41.3,31.2079933773895)) ;
#14567=CARTESIAN_POINT('Origin',(72.2463448275862,41.3,40.6079933773895)) ;
#14568=CARTESIAN_POINT('',(72.2463448275862,41.3,40.6079933773895)) ;
#14569=CARTESIAN_POINT('',(72.2463448275862,41.3,40.6079933773895)) ;
#14570=CARTESIAN_POINT('',(72.2463448275862,44.3,40.6079933773895)) ;
#14571=CARTESIAN_POINT('',(72.2463448275862,44.3,40.6079933773895)) ;
#14572=CARTESIAN_POINT('',(72.2463448275862,41.3,40.6079933773895)) ;
#14573=CARTESIAN_POINT('Origin',(72.,41.3,44.4)) ;
#14574=CARTESIAN_POINT('Origin',(72.,41.3,44.4)) ;
#14575=CARTESIAN_POINT('Origin',(72.,44.3,44.4)) ;
#14576=CARTESIAN_POINT('Origin',(-0.347494773488863,44.3,39.7)) ;
#14577=CARTESIAN_POINT('Origin',(-0.347494773488863,41.3,39.7)) ;
#18724=UNCERTAINTY_MEASURE_WITH_UNIT(LENGTH_MEASURE(0.01),#18758,
'DISTANCE_ACCURACY_VALUE',
'Maximum model space distance between geometric entities at asserted c
onnectivities') ;
#18738=UNCERTAINTY_MEASURE_WITH_UNIT(LENGTH_MEASURE(0.01),#18758,
'DISTANCE_ACCURACY_VALUE',
'Maximum model space distance between geometric entities at asserted c
onnectivities') ;
#18743=(
GEOMETRIC_REPRESENTATION_CONTEXT(3)
GLOBAL_UNCERTAINTY_ASSIGNED_CONTEXT((#18724))
GLOBAL_UNIT_ASSIGNED_CONTEXT((#18758,#18760,#18761))
REPRESENTATION_CONTEXT('','3D')
) ;
#18757=(
GEOMETRIC_REPRESENTATION_CONTEXT(3)
GLOBAL_UNCERTAINTY_ASSIGNED_CONTEXT((#18738))
GLOBAL_UNIT_ASSIGNED_CONTEXT((#18758,#18760,#18761))
REPRESENTATION_CONTEXT('','3D')
) ;
#18758=(
LENGTH_UNIT()
NAMED_UNIT(*)
SI_UNIT(.MILLI.,.METRE.)
) ;
#18760=(
NAMED_UNIT(*)
PLANE_ANGLE_UNIT()
SI_UNIT($,.RADIAN.)
) ;
#18761=(
NAMED_UNIT(*)
SI_UNIT($,.STERADIAN.)
SOLID_ANGLE_UNIT()
) ;
#18766=SHAPE_DEFINITION_REPRESENTATION(#18784,#18860) ;
#18784=PRODUCT_DEFINITION_SHAPE('',$,#18879) ;
#18860=SHAPE_REPRESENTATION('',(#10025),#18743) ;
#18874=PRODUCT_DEFINITION_CONTEXT('part definition',#18930,'design') ;
#18879=PRODUCT_DEFINITION('Inner Scissor Arm Frame',
'Inner Scissor Arm Frame',#18897,#18874) ;
#18897=PRODUCT_DEFINITION_FORMATION('',$,#18936) ;
#18930=APPLICATION_CONTEXT(
'Core Data for Automotive Mechanical Design Process') ;
#18931=PRODUCT_CONTEXT('part definition',#18930,'mechanical') ;
#18936=PRODUCT('Inner Scissor Arm Frame','Inner Scissor Arm Frame',$,(#18931)) ;
#18954=PRESENTATION_STYLE_ASSIGNMENT((#18972)) ;
#18972=SURFACE_STYLE_USAGE(.BOTH.,#18990) ;
#18990=SURFACE_SIDE_STYLE('',(#19008)) ;
#19008=SURFACE_STYLE_FILL_AREA(#19026) ;
#19026=FILL_AREA_STYLE(
'MAS-253 Metallic Sheet - Inner Scissor Arm Frame',(#19044)) ;
#19044=FILL_AREA_STYLE_COLOUR(
'MAS-253 Metallic Sheet - Inner Scissor Arm Frame',#19062) ;
#19062=COLOUR_RGB('MAS-253 Metallic Sheet - Inner Scissor Arm Frame', 0.72549020, 0.75294118, 0.79215686) ;
ENDSEC;
END-ISO-10303-21;
